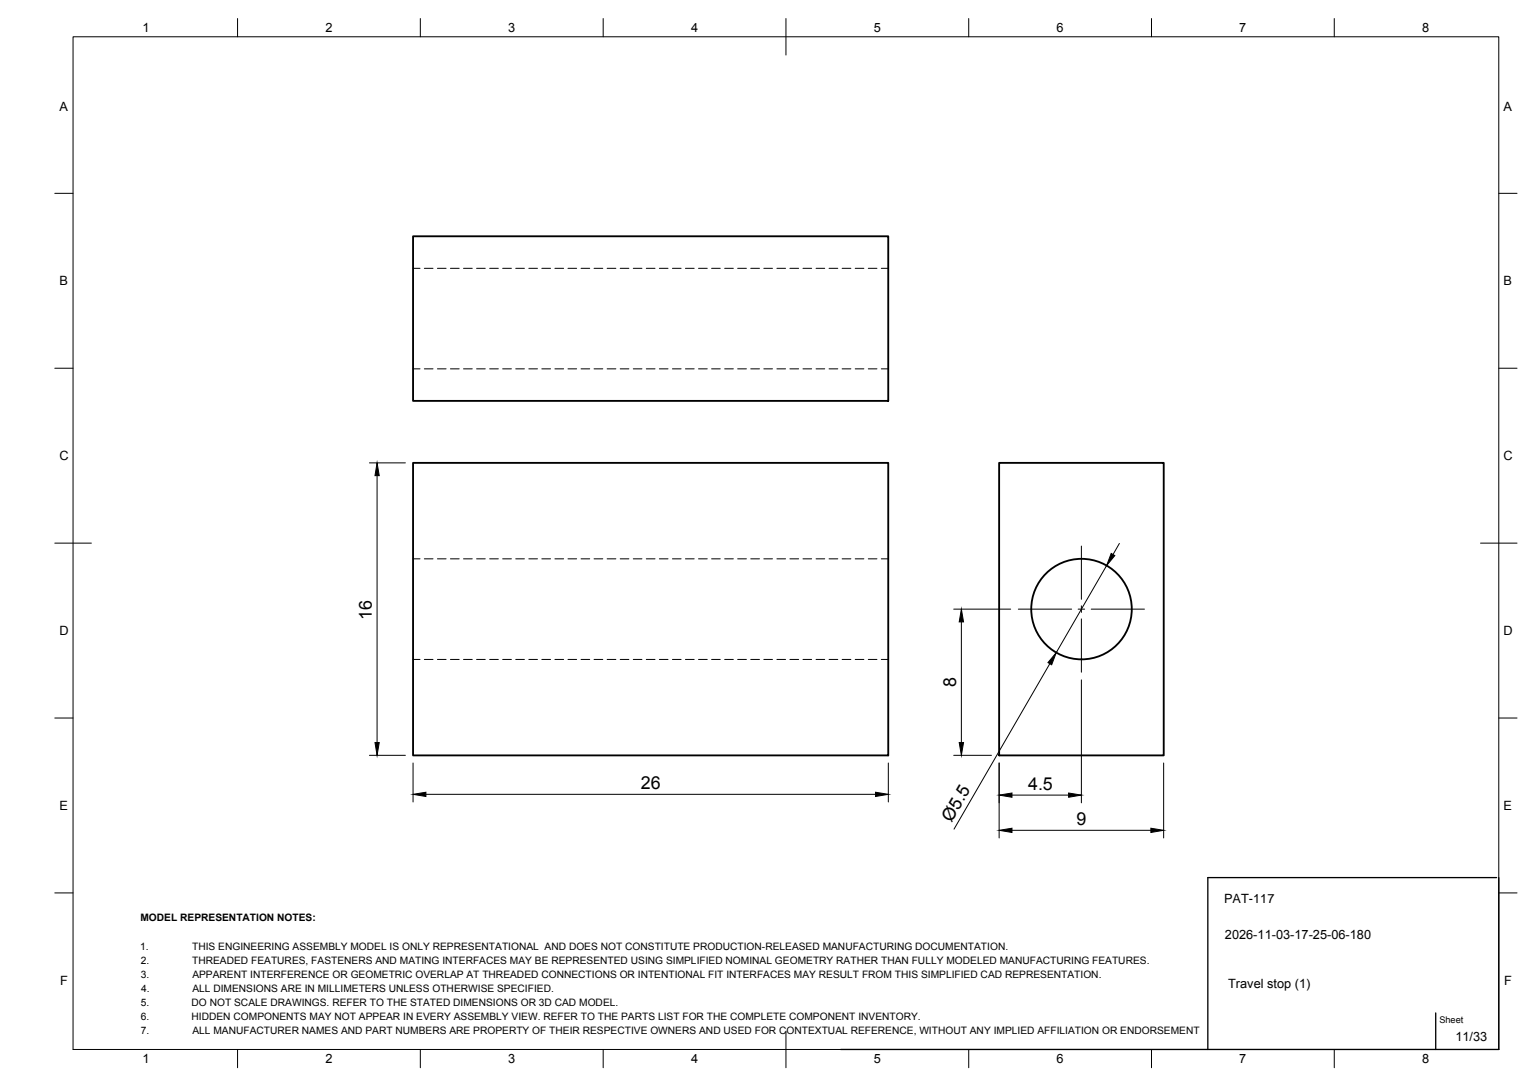
ISO-10303-21;
HEADER;
/* Generated by software containing ST-Developer
 * from STEP Tools, Inc. (www.steptools.com) 
 */

FILE_DESCRIPTION(
/* description */ ('Counterbalanced vertical column'),
/* implementation_level */ '2;1');

FILE_NAME(
/* name */ 'Travel stop (1).step',
/* time_stamp */ '2026-10-29T16:47:22-07:00',
/* author */ (''),
/* organization */ (''),
/* preprocessor_version */ 'ST-DEVELOPER v20.2',
/* originating_system */ 'Autodesk Translation Framework v15.17.0.0',
/* authorisation */ '');

FILE_SCHEMA (('AUTOMOTIVE_DESIGN { 1 0 10303 214 3 1 1 }'));
ENDSEC;

DATA;
#10=MECHANICAL_DESIGN_GEOMETRIC_PRESENTATION_REPRESENTATION('',(#356),#15040);
#286=SHAPE_REPRESENTATION_RELATIONSHIP('SRR','None',#15190,#321);
#321=ADVANCED_BREP_SHAPE_REPRESENTATION('',(#391),#15009);
#356=STYLED_ITEM('',(#15443),#391);
#391=MANIFOLD_SOLID_BREP('Body1',#7079);
#442=FACE_BOUND('',#1319,.T.);
#443=FACE_BOUND('',#1322,.T.);
#575=PLANE('',#7599);
#576=PLANE('',#7600);
#577=PLANE('',#7601);
#578=PLANE('',#7602);
#579=PLANE('',#7603);
#580=PLANE('',#7604);
#885=FACE_OUTER_BOUND('',#1316,.T.);
#886=FACE_OUTER_BOUND('',#1317,.T.);
#887=FACE_OUTER_BOUND('',#1318,.T.);
#888=FACE_OUTER_BOUND('',#1320,.T.);
#889=FACE_OUTER_BOUND('',#1321,.T.);
#890=FACE_OUTER_BOUND('',#1323,.T.);
#891=FACE_OUTER_BOUND('',#1324,.T.);
#1316=EDGE_LOOP('',(#5046,#5047,#5048,#5049));
#1317=EDGE_LOOP('',(#5050,#5051,#5052,#5053));
#1318=EDGE_LOOP('',(#5054,#5055,#5056,#5057));
#1319=EDGE_LOOP('',(#5058));
#1320=EDGE_LOOP('',(#5059,#5060,#5061,#5062));
#1321=EDGE_LOOP('',(#5063,#5064,#5065,#5066));
#1322=EDGE_LOOP('',(#5067));
#1323=EDGE_LOOP('',(#5068,#5069,#5070,#5071));
#1324=EDGE_LOOP('',(#5072,#5073,#5074,#5075));
#1850=LINE('',#10625,#2521);
#1851=LINE('',#10630,#2522);
#1852=LINE('',#10632,#2523);
#1853=LINE('',#10634,#2524);
#1854=LINE('',#10635,#2525);
#1855=LINE('',#10638,#2526);
#1856=LINE('',#10640,#2527);
#1857=LINE('',#10641,#2528);
#1858=LINE('',#10644,#2529);
#1859=LINE('',#10646,#2530);
#1860=LINE('',#10647,#2531);
#1861=LINE('',#10649,#2532);
#1862=LINE('',#10650,#2533);
#2521=VECTOR('',#8520,0.274999999999999);
#2522=VECTOR('',#8525,1.);
#2523=VECTOR('',#8526,1.);
#2524=VECTOR('',#8527,1.);
#2525=VECTOR('',#8528,1.);
#2526=VECTOR('',#8531,1.);
#2527=VECTOR('',#8532,1.);
#2528=VECTOR('',#8533,1.);
#2529=VECTOR('',#8536,1.);
#2530=VECTOR('',#8537,1.);
#2531=VECTOR('',#8538,1.);
#2532=VECTOR('',#8541,1.);
#2533=VECTOR('',#8542,1.);
#3123=CIRCLE('',#7597,0.274999999999999);
#3124=CIRCLE('',#7598,0.274999999999999);
#3392=VERTEX_POINT('',#10622);
#3393=VERTEX_POINT('',#10624);
#3394=VERTEX_POINT('',#10628);
#3395=VERTEX_POINT('',#10629);
#3396=VERTEX_POINT('',#10631);
#3397=VERTEX_POINT('',#10633);
#3398=VERTEX_POINT('',#10637);
#3399=VERTEX_POINT('',#10639);
#3400=VERTEX_POINT('',#10643);
#3401=VERTEX_POINT('',#10645);
#4024=EDGE_CURVE('',#3392,#3392,#3123,.T.);
#4025=EDGE_CURVE('',#3392,#3393,#1850,.T.);
#4026=EDGE_CURVE('',#3393,#3393,#3124,.T.);
#4027=EDGE_CURVE('',#3394,#3395,#1851,.T.);
#4028=EDGE_CURVE('',#3395,#3396,#1852,.T.);
#4029=EDGE_CURVE('',#3397,#3396,#1853,.T.);
#4030=EDGE_CURVE('',#3394,#3397,#1854,.T.);
#4031=EDGE_CURVE('',#3398,#3394,#1855,.T.);
#4032=EDGE_CURVE('',#3399,#3397,#1856,.T.);
#4033=EDGE_CURVE('',#3398,#3399,#1857,.T.);
#4034=EDGE_CURVE('',#3400,#3398,#1858,.T.);
#4035=EDGE_CURVE('',#3401,#3399,#1859,.T.);
#4036=EDGE_CURVE('',#3400,#3401,#1860,.T.);
#4037=EDGE_CURVE('',#3395,#3400,#1861,.T.);
#4038=EDGE_CURVE('',#3396,#3401,#1862,.T.);
#5046=ORIENTED_EDGE('',*,*,#4024,.F.);
#5047=ORIENTED_EDGE('',*,*,#4025,.T.);
#5048=ORIENTED_EDGE('',*,*,#4026,.F.);
#5049=ORIENTED_EDGE('',*,*,#4025,.F.);
#5050=ORIENTED_EDGE('',*,*,#4027,.T.);
#5051=ORIENTED_EDGE('',*,*,#4028,.T.);
#5052=ORIENTED_EDGE('',*,*,#4029,.F.);
#5053=ORIENTED_EDGE('',*,*,#4030,.F.);
#5054=ORIENTED_EDGE('',*,*,#4031,.T.);
#5055=ORIENTED_EDGE('',*,*,#4030,.T.);
#5056=ORIENTED_EDGE('',*,*,#4032,.F.);
#5057=ORIENTED_EDGE('',*,*,#4033,.F.);
#5058=ORIENTED_EDGE('',*,*,#4026,.T.);
#5059=ORIENTED_EDGE('',*,*,#4034,.T.);
#5060=ORIENTED_EDGE('',*,*,#4033,.T.);
#5061=ORIENTED_EDGE('',*,*,#4035,.F.);
#5062=ORIENTED_EDGE('',*,*,#4036,.F.);
#5063=ORIENTED_EDGE('',*,*,#4037,.T.);
#5064=ORIENTED_EDGE('',*,*,#4036,.T.);
#5065=ORIENTED_EDGE('',*,*,#4038,.F.);
#5066=ORIENTED_EDGE('',*,*,#4028,.F.);
#5067=ORIENTED_EDGE('',*,*,#4024,.T.);
#5068=ORIENTED_EDGE('',*,*,#4038,.T.);
#5069=ORIENTED_EDGE('',*,*,#4035,.T.);
#5070=ORIENTED_EDGE('',*,*,#4032,.T.);
#5071=ORIENTED_EDGE('',*,*,#4029,.T.);
#5072=ORIENTED_EDGE('',*,*,#4037,.F.);
#5073=ORIENTED_EDGE('',*,*,#4027,.F.);
#5074=ORIENTED_EDGE('',*,*,#4031,.F.);
#5075=ORIENTED_EDGE('',*,*,#4034,.F.);
#6589=CYLINDRICAL_SURFACE('',#7596,0.274999999999999);
#6727=ADVANCED_FACE('',(#885),#6589,.F.);
#6728=ADVANCED_FACE('',(#886),#575,.T.);
#6729=ADVANCED_FACE('',(#887,#442),#576,.T.);
#6730=ADVANCED_FACE('',(#888),#577,.T.);
#6731=ADVANCED_FACE('',(#889,#443),#578,.T.);
#6732=ADVANCED_FACE('',(#890),#579,.T.);
#6733=ADVANCED_FACE('',(#891),#580,.F.);
#7079=CLOSED_SHELL('',(#6727,#6728,#6729,#6730,#6731,#6732,#6733));
#7595=AXIS2_PLACEMENT_3D('',#10620,#8514,#8515);
#7596=AXIS2_PLACEMENT_3D('',#10621,#8516,#8517);
#7597=AXIS2_PLACEMENT_3D('',#10623,#8518,#8519);
#7598=AXIS2_PLACEMENT_3D('',#10626,#8521,#8522);
#7599=AXIS2_PLACEMENT_3D('',#10627,#8523,#8524);
#7600=AXIS2_PLACEMENT_3D('',#10636,#8529,#8530);
#7601=AXIS2_PLACEMENT_3D('',#10642,#8534,#8535);
#7602=AXIS2_PLACEMENT_3D('',#10648,#8539,#8540);
#7603=AXIS2_PLACEMENT_3D('',#10651,#8543,#8544);
#7604=AXIS2_PLACEMENT_3D('',#10652,#8545,#8546);
#8514=DIRECTION('axis',(0.,0.,1.));
#8515=DIRECTION('refdir',(1.,0.,0.));
#8516=DIRECTION('center_axis',(1.,0.,0.));
#8517=DIRECTION('ref_axis',(0.,0.,-1.));
#8518=DIRECTION('center_axis',(1.,0.,0.));
#8519=DIRECTION('ref_axis',(0.,0.,-1.));
#8520=DIRECTION('',(1.,0.,0.));
#8521=DIRECTION('center_axis',(-1.,0.,0.));
#8522=DIRECTION('ref_axis',(0.,0.,-1.));
#8523=DIRECTION('center_axis',(0.,1.,0.));
#8524=DIRECTION('ref_axis',(-1.,0.,0.));
#8525=DIRECTION('',(-1.,0.,0.));
#8526=DIRECTION('',(0.,0.,1.));
#8527=DIRECTION('',(-1.,0.,0.));
#8528=DIRECTION('',(0.,0.,1.));
#8529=DIRECTION('center_axis',(1.,0.,0.));
#8530=DIRECTION('ref_axis',(0.,1.,0.));
#8531=DIRECTION('',(0.,1.,0.));
#8532=DIRECTION('',(0.,1.,0.));
#8533=DIRECTION('',(0.,0.,1.));
#8534=DIRECTION('center_axis',(0.,-1.,0.));
#8535=DIRECTION('ref_axis',(1.,0.,0.));
#8536=DIRECTION('',(1.,0.,0.));
#8537=DIRECTION('',(1.,0.,0.));
#8538=DIRECTION('',(0.,0.,1.));
#8539=DIRECTION('center_axis',(-1.,0.,0.));
#8540=DIRECTION('ref_axis',(0.,-1.,0.));
#8541=DIRECTION('',(0.,-1.,0.));
#8542=DIRECTION('',(0.,-1.,0.));
#8543=DIRECTION('center_axis',(0.,0.,1.));
#8544=DIRECTION('ref_axis',(1.,0.,0.));
#8545=DIRECTION('center_axis',(0.,0.,1.));
#8546=DIRECTION('ref_axis',(1.,0.,0.));
#10620=CARTESIAN_POINT('',(0.,0.,0.));
#10621=CARTESIAN_POINT('Origin',(-1.5,2.,33.45));
#10622=CARTESIAN_POINT('',(-1.4,2.,33.725));
#10623=CARTESIAN_POINT('Origin',(-1.4,2.,33.45));
#10624=CARTESIAN_POINT('',(1.2,2.,33.725));
#10625=CARTESIAN_POINT('',(-1.5,2.,33.725));
#10626=CARTESIAN_POINT('Origin',(1.2,2.,33.45));
#10627=CARTESIAN_POINT('Origin',(1.2,2.8,33.));
#10628=CARTESIAN_POINT('',(1.2,2.8,33.));
#10629=CARTESIAN_POINT('',(-1.4,2.8,33.));
#10630=CARTESIAN_POINT('',(1.2,2.8,33.));
#10631=CARTESIAN_POINT('',(-1.4,2.8,33.9));
#10632=CARTESIAN_POINT('',(-1.4,2.8,33.));
#10633=CARTESIAN_POINT('',(1.2,2.8,33.9));
#10634=CARTESIAN_POINT('',(1.2,2.8,33.9));
#10635=CARTESIAN_POINT('',(1.2,2.8,33.));
#10636=CARTESIAN_POINT('Origin',(1.2,1.2,33.));
#10637=CARTESIAN_POINT('',(1.2,1.2,33.));
#10638=CARTESIAN_POINT('',(1.2,1.2,33.));
#10639=CARTESIAN_POINT('',(1.2,1.2,33.9));
#10640=CARTESIAN_POINT('',(1.2,1.2,33.9));
#10641=CARTESIAN_POINT('',(1.2,1.2,33.));
#10642=CARTESIAN_POINT('Origin',(-1.4,1.2,33.));
#10643=CARTESIAN_POINT('',(-1.4,1.2,33.));
#10644=CARTESIAN_POINT('',(-1.4,1.2,33.));
#10645=CARTESIAN_POINT('',(-1.4,1.2,33.9));
#10646=CARTESIAN_POINT('',(-1.4,1.2,33.9));
#10647=CARTESIAN_POINT('',(-1.4,1.2,33.));
#10648=CARTESIAN_POINT('Origin',(-1.4,2.8,33.));
#10649=CARTESIAN_POINT('',(-1.4,2.8,33.));
#10650=CARTESIAN_POINT('',(-1.4,2.8,33.9));
#10651=CARTESIAN_POINT('Origin',(-0.1,2.,33.9));
#10652=CARTESIAN_POINT('Origin',(-0.1,2.,33.));
#14969=UNCERTAINTY_MEASURE_WITH_UNIT(LENGTH_MEASURE(0.001),#15041,
'DISTANCE_ACCURACY_VALUE',
'Maximum model space distance between geometric entities at asserted c
onnectivities');
#15000=UNCERTAINTY_MEASURE_WITH_UNIT(LENGTH_MEASURE(0.001),#15041,
'DISTANCE_ACCURACY_VALUE',
'Maximum model space distance between geometric entities at asserted c
onnectivities');
#15009=(
GEOMETRIC_REPRESENTATION_CONTEXT(3)
GLOBAL_UNCERTAINTY_ASSIGNED_CONTEXT((#14969))
GLOBAL_UNIT_ASSIGNED_CONTEXT((#15041,#15043,#15044))
REPRESENTATION_CONTEXT('','3D')
);
#15040=(
GEOMETRIC_REPRESENTATION_CONTEXT(3)
GLOBAL_UNCERTAINTY_ASSIGNED_CONTEXT((#15000))
GLOBAL_UNIT_ASSIGNED_CONTEXT((#15041,#15043,#15044))
REPRESENTATION_CONTEXT('','3D')
);
#15041=(
LENGTH_UNIT()
NAMED_UNIT(*)
SI_UNIT(.CENTI.,.METRE.)
);
#15043=(
NAMED_UNIT(*)
PLANE_ANGLE_UNIT()
SI_UNIT($,.RADIAN.)
);
#15044=(
NAMED_UNIT(*)
SI_UNIT($,.STERADIAN.)
SOLID_ANGLE_UNIT()
);
#15053=SHAPE_DEFINITION_REPRESENTATION(#15092,#15190);
#15092=PRODUCT_DEFINITION_SHAPE('',$,#15230);
#15190=SHAPE_REPRESENTATION('',(#7595),#15009);
#15221=PRODUCT_DEFINITION_CONTEXT('part definition',#15340,'design');
#15230=PRODUCT_DEFINITION('Travel stop (1)','Travel stop (1)',#15269,#15221);
#15269=PRODUCT_DEFINITION_FORMATION('',$,#15350);
#15340=APPLICATION_CONTEXT(
'Core Data for Automotive Mechanical Design Process');
#15341=PRODUCT_CONTEXT('part definition',#15340,'mechanical');
#15350=PRODUCT('Travel stop (1)','Travel stop (1)','Travel stop (1)',(#15341));
#15437=COLOUR_RGB('Light Blue',0.38,0.62,0.78);
#15438=FILL_AREA_STYLE_COLOUR('',#15437);
#15439=FILL_AREA_STYLE('',(#15438));
#15440=SURFACE_STYLE_FILL_AREA(#15439);
#15441=SURFACE_SIDE_STYLE('',(#15440));
#15442=SURFACE_STYLE_USAGE(.BOTH.,#15441);
#15443=PRESENTATION_STYLE_ASSIGNMENT((#15442));
ENDSEC;
END-ISO-10303-21;
